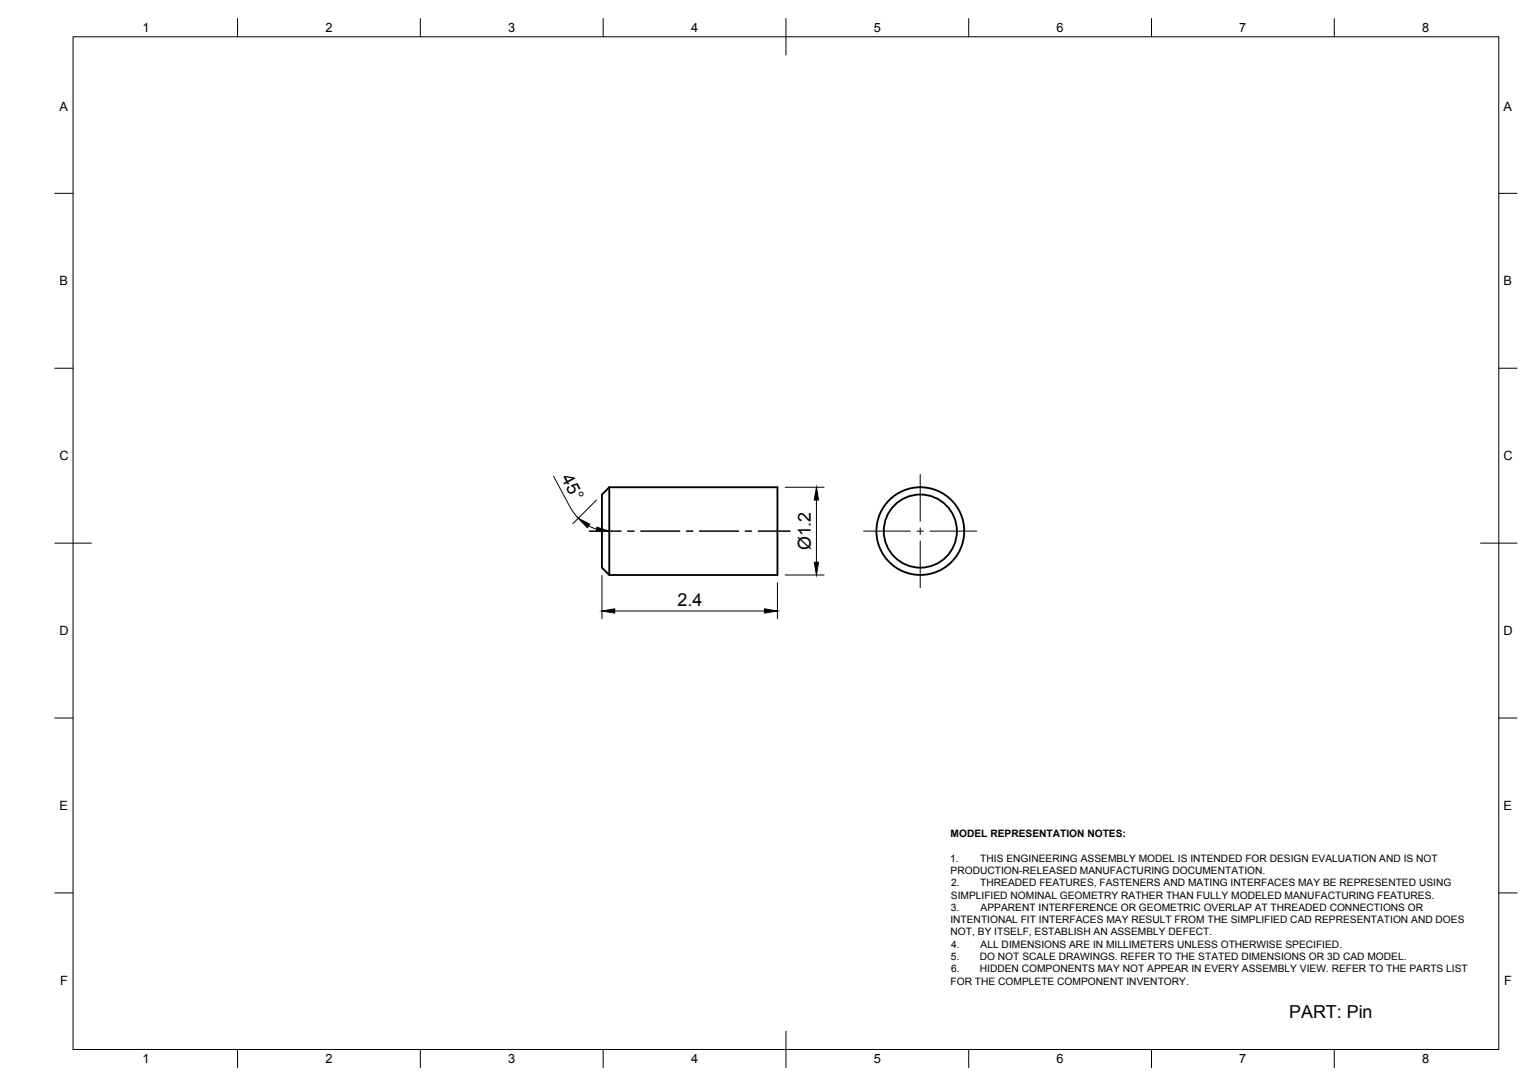
ISO-10303-21;
HEADER;
/* Generated by software containing ST-Developer
 * from STEP Tools, Inc. (www.steptools.com) 
 */

FILE_DESCRIPTION(
/* description */ (''),
/* implementation_level */ '2;1');

FILE_NAME(
/* name */ 'Pin.step',
/* time_stamp */ '2026-10-05T00:51:14-07:00',
/* author */ (''),
/* organization */ (''),
/* preprocessor_version */ 'ST-DEVELOPER v20.2',
/* originating_system */ 'Autodesk Translation Framework v15.15.0.0',
/* authorisation */ '');

FILE_SCHEMA (('AUTOMOTIVE_DESIGN { 1 0 10303 214 3 1 1 }'));
ENDSEC;

DATA;
#10=MECHANICAL_DESIGN_GEOMETRIC_PRESENTATION_REPRESENTATION('',(#394),#4613);
#66=CONICAL_SURFACE('',#1887,0.550000000000002,0.785398163397437);
#130=PLANE('',#1892);
#131=PLANE('',#1893);
#246=LINE('',#4578,#329);
#247=LINE('',#4582,#330);
#329=VECTOR('',#2379,0.550000000000002);
#330=VECTOR('',#2384,0.600000000000001);
#370=CYLINDRICAL_SURFACE('',#1890,0.600000000000001);
#378=SHAPE_REPRESENTATION_RELATIONSHIP('SRR','None',#4652,#386);
#386=ADVANCED_BREP_SHAPE_REPRESENTATION('',(#402),#4612);
#394=STYLED_ITEM('',(#4697),#402);
#402=MANIFOLD_SOLID_BREP('Body1',#1601);
#505=FACE_OUTER_BOUND('',#635,.T.);
#506=FACE_OUTER_BOUND('',#636,.T.);
#507=FACE_OUTER_BOUND('',#637,.T.);
#508=FACE_OUTER_BOUND('',#638,.T.);
#635=EDGE_LOOP('',(#1477,#1478,#1479,#1480));
#636=EDGE_LOOP('',(#1481,#1482,#1483,#1484));
#637=EDGE_LOOP('',(#1485));
#638=EDGE_LOOP('',(#1486));
#728=CIRCLE('',#1888,0.600000000000001);
#729=CIRCLE('',#1889,0.500000000000003);
#730=CIRCLE('',#1891,0.600000000000001);
#860=VERTEX_POINT('',#4575);
#861=VERTEX_POINT('',#4577);
#862=VERTEX_POINT('',#4581);
#1066=EDGE_CURVE('',#860,#860,#728,.T.);
#1067=EDGE_CURVE('',#860,#861,#246,.T.);
#1068=EDGE_CURVE('',#861,#861,#729,.T.);
#1069=EDGE_CURVE('',#860,#862,#247,.T.);
#1070=EDGE_CURVE('',#862,#862,#730,.T.);
#1477=ORIENTED_EDGE('',*,*,#1066,.T.);
#1478=ORIENTED_EDGE('',*,*,#1067,.T.);
#1479=ORIENTED_EDGE('',*,*,#1068,.T.);
#1480=ORIENTED_EDGE('',*,*,#1067,.F.);
#1481=ORIENTED_EDGE('',*,*,#1066,.F.);
#1482=ORIENTED_EDGE('',*,*,#1069,.T.);
#1483=ORIENTED_EDGE('',*,*,#1070,.T.);
#1484=ORIENTED_EDGE('',*,*,#1069,.F.);
#1485=ORIENTED_EDGE('',*,*,#1068,.F.);
#1486=ORIENTED_EDGE('',*,*,#1070,.F.);
#1590=ADVANCED_FACE('',(#505),#66,.T.);
#1591=ADVANCED_FACE('',(#506),#370,.T.);
#1592=ADVANCED_FACE('',(#507),#130,.T.);
#1593=ADVANCED_FACE('',(#508),#131,.F.);
#1601=CLOSED_SHELL('',(#1590,#1591,#1592,#1593));
#1886=AXIS2_PLACEMENT_3D('',#4573,#2373,#2374);
#1887=AXIS2_PLACEMENT_3D('',#4574,#2375,#2376);
#1888=AXIS2_PLACEMENT_3D('',#4576,#2377,#2378);
#1889=AXIS2_PLACEMENT_3D('',#4579,#2380,#2381);
#1890=AXIS2_PLACEMENT_3D('',#4580,#2382,#2383);
#1891=AXIS2_PLACEMENT_3D('',#4583,#2385,#2386);
#1892=AXIS2_PLACEMENT_3D('',#4584,#2387,#2388);
#1893=AXIS2_PLACEMENT_3D('',#4585,#2389,#2390);
#2373=DIRECTION('axis',(0.,0.,1.));
#2374=DIRECTION('refdir',(1.,0.,0.));
#2375=DIRECTION('center_axis',(0.,0.,-1.));
#2376=DIRECTION('ref_axis',(1.,0.,0.));
#2377=DIRECTION('center_axis',(0.,0.,1.));
#2378=DIRECTION('ref_axis',(1.,0.,0.));
#2379=DIRECTION('',(0.707106781186539,-8.65956056235483E-17,0.707106781186556));
#2380=DIRECTION('center_axis',(0.,0.,-1.));
#2381=DIRECTION('ref_axis',(1.,0.,0.));
#2382=DIRECTION('center_axis',(0.,0.,1.));
#2383=DIRECTION('ref_axis',(1.,0.,0.));
#2384=DIRECTION('',(0.,0.,-1.));
#2385=DIRECTION('center_axis',(0.,0.,1.));
#2386=DIRECTION('ref_axis',(1.,0.,0.));
#2387=DIRECTION('center_axis',(0.,0.,1.));
#2388=DIRECTION('ref_axis',(1.,0.,0.));
#2389=DIRECTION('center_axis',(0.,0.,1.));
#2390=DIRECTION('ref_axis',(1.,0.,0.));
#4573=CARTESIAN_POINT('',(0.,0.,0.));
#4574=CARTESIAN_POINT('Origin',(-25.2637346688979,0.,2.35));
#4575=CARTESIAN_POINT('',(-25.8637346688979,-7.34788079488413E-17,2.3));
#4576=CARTESIAN_POINT('Origin',(-25.2637346688979,0.,2.3));
#4577=CARTESIAN_POINT('',(-25.7637346688979,6.1232339957368E-17,2.4));
#4578=CARTESIAN_POINT('',(-25.8137346688979,6.73555739531047E-17,2.35));
#4579=CARTESIAN_POINT('Origin',(-25.2637346688979,0.,2.4));
#4580=CARTESIAN_POINT('Origin',(-25.2637346688979,0.,0.));
#4581=CARTESIAN_POINT('',(-25.8637346688979,-7.34788079488413E-17,0.));
#4582=CARTESIAN_POINT('',(-25.8637346688979,-7.34788079488413E-17,0.));
#4583=CARTESIAN_POINT('Origin',(-25.2637346688979,0.,0.));
#4584=CARTESIAN_POINT('Origin',(-25.2637346688979,0.,2.4));
#4585=CARTESIAN_POINT('Origin',(-25.2637346688979,0.,0.));
#4602=UNCERTAINTY_MEASURE_WITH_UNIT(LENGTH_MEASURE(0.01),#4614,
'DISTANCE_ACCURACY_VALUE',
'Maximum model space distance between geometric entities at asserted c
onnectivities');
#4603=UNCERTAINTY_MEASURE_WITH_UNIT(LENGTH_MEASURE(0.01),#4614,
'DISTANCE_ACCURACY_VALUE',
'Maximum model space distance between geometric entities at asserted c
onnectivities');
#4612=(
GEOMETRIC_REPRESENTATION_CONTEXT(3)
GLOBAL_UNCERTAINTY_ASSIGNED_CONTEXT((#4602))
GLOBAL_UNIT_ASSIGNED_CONTEXT((#4614,#4616,#4617))
REPRESENTATION_CONTEXT('','3D')
);
#4613=(
GEOMETRIC_REPRESENTATION_CONTEXT(3)
GLOBAL_UNCERTAINTY_ASSIGNED_CONTEXT((#4603))
GLOBAL_UNIT_ASSIGNED_CONTEXT((#4614,#4616,#4617))
REPRESENTATION_CONTEXT('','3D')
);
#4614=(
LENGTH_UNIT()
NAMED_UNIT(*)
SI_UNIT(.MILLI.,.METRE.)
);
#4616=(
NAMED_UNIT(*)
PLANE_ANGLE_UNIT()
SI_UNIT($,.RADIAN.)
);
#4617=(
NAMED_UNIT(*)
SI_UNIT($,.STERADIAN.)
SOLID_ANGLE_UNIT()
);
#4626=SHAPE_DEFINITION_REPRESENTATION(#4635,#4652);
#4635=PRODUCT_DEFINITION_SHAPE('',$,#4662);
#4652=SHAPE_REPRESENTATION('',(#1886),#4612);
#4653=PRODUCT_DEFINITION_CONTEXT('part definition',#4682,'design');
#4662=PRODUCT_DEFINITION('Pin','Pin',#4671,#4653);
#4671=PRODUCT_DEFINITION_FORMATION('',$,#4692);
#4682=APPLICATION_CONTEXT(
'Core Data for Automotive Mechanical Design Process');
#4683=PRODUCT_CONTEXT('part definition',#4682,'mechanical');
#4692=PRODUCT('Pin','Pin',$,(#4683));
#4697=PRESENTATION_STYLE_ASSIGNMENT((#4702));
#4702=SURFACE_STYLE_USAGE(.BOTH.,#4707);
#4707=SURFACE_SIDE_STYLE('',(#4712));
#4712=SURFACE_STYLE_FILL_AREA(#4717);
#4717=FILL_AREA_STYLE('Opaque(160,160,160)',(#4722));
#4722=FILL_AREA_STYLE_COLOUR('Opaque(160,160,160)',#4727);
#4727=COLOUR_RGB('Opaque(160,160,160)', 0.66274510, 0.83137255, 0.94901961);
ENDSEC;
END-ISO-10303-21;
